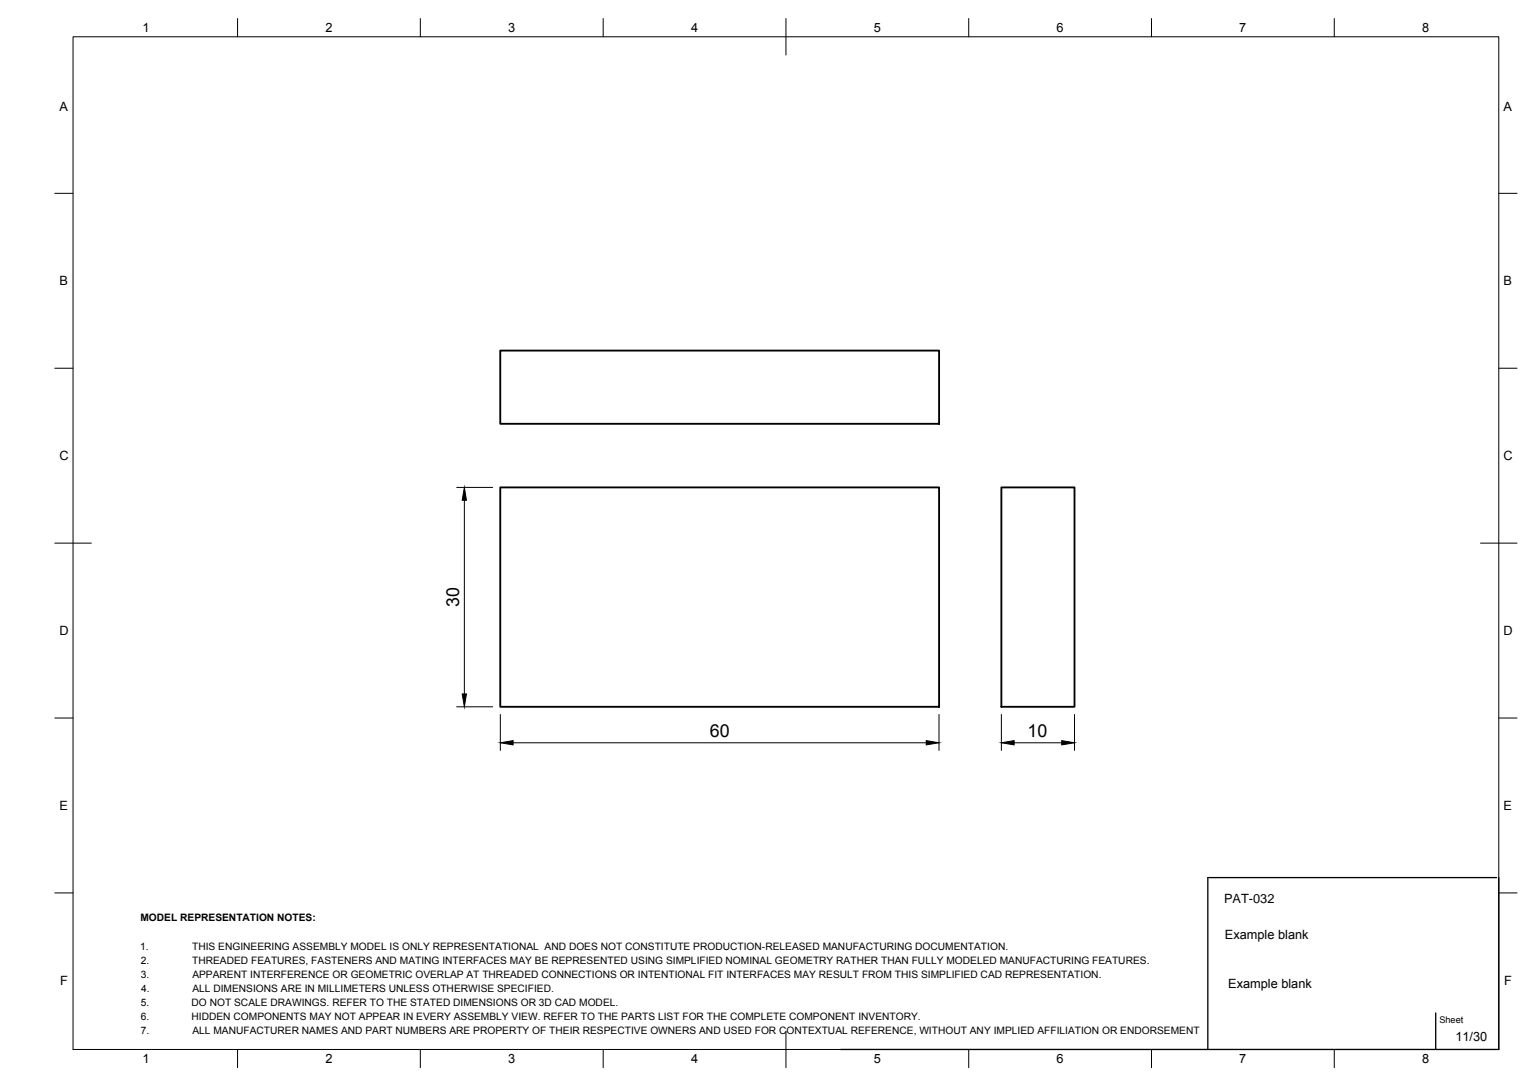
ISO-10303-21;
HEADER;
/* Generated by software containing ST-Developer
 * from STEP Tools, Inc. (www.steptools.com) 
 */

FILE_DESCRIPTION(
/* description */ ('Drill jig with bushing plate'),
/* implementation_level */ '2;1');

FILE_NAME(
/* name */ 'Example blank.step',
/* time_stamp */ '2026-10-27T10:51:08-07:00',
/* author */ (''),
/* organization */ (''),
/* preprocessor_version */ 'ST-DEVELOPER v20.2',
/* originating_system */ 'Autodesk Translation Framework v15.17.0.0',
/* authorisation */ '');

FILE_SCHEMA (('AUTOMOTIVE_DESIGN { 1 0 10303 214 3 1 1 }'));
ENDSEC;

DATA;
#10=MECHANICAL_DESIGN_GEOMETRIC_PRESENTATION_REPRESENTATION('',(#229),#6638);
#181=SHAPE_REPRESENTATION_RELATIONSHIP('SRR','None',#6745,#205);
#205=ADVANCED_BREP_SHAPE_REPRESENTATION('',(#253),#6618);
#229=STYLED_ITEM('',(#6929),#253);
#253=MANIFOLD_SOLID_BREP('Body1',#3596);
#399=PLANE('',#3997);
#400=PLANE('',#3998);
#401=PLANE('',#3999);
#402=PLANE('',#4000);
#403=PLANE('',#4001);
#404=PLANE('',#4002);
#556=FACE_OUTER_BOUND('',#811,.T.);
#557=FACE_OUTER_BOUND('',#812,.T.);
#558=FACE_OUTER_BOUND('',#813,.T.);
#559=FACE_OUTER_BOUND('',#814,.T.);
#560=FACE_OUTER_BOUND('',#815,.T.);
#561=FACE_OUTER_BOUND('',#816,.T.);
#811=EDGE_LOOP('',(#2665,#2666,#2667,#2668));
#812=EDGE_LOOP('',(#2669,#2670,#2671,#2672));
#813=EDGE_LOOP('',(#2673,#2674,#2675,#2676));
#814=EDGE_LOOP('',(#2677,#2678,#2679,#2680));
#815=EDGE_LOOP('',(#2681,#2682,#2683,#2684));
#816=EDGE_LOOP('',(#2685,#2686,#2687,#2688));
#1092=LINE('',#5743,#1353);
#1093=LINE('',#5745,#1354);
#1094=LINE('',#5747,#1355);
#1095=LINE('',#5748,#1356);
#1096=LINE('',#5751,#1357);
#1097=LINE('',#5753,#1358);
#1098=LINE('',#5754,#1359);
#1099=LINE('',#5757,#1360);
#1100=LINE('',#5759,#1361);
#1101=LINE('',#5760,#1362);
#1102=LINE('',#5762,#1363);
#1103=LINE('',#5763,#1364);
#1353=VECTOR('',#4625,1.);
#1354=VECTOR('',#4626,1.);
#1355=VECTOR('',#4627,1.);
#1356=VECTOR('',#4628,1.);
#1357=VECTOR('',#4631,1.);
#1358=VECTOR('',#4632,1.);
#1359=VECTOR('',#4633,1.);
#1360=VECTOR('',#4636,1.);
#1361=VECTOR('',#4637,1.);
#1362=VECTOR('',#4638,1.);
#1363=VECTOR('',#4641,1.);
#1364=VECTOR('',#4642,1.);
#1796=VERTEX_POINT('',#5741);
#1797=VERTEX_POINT('',#5742);
#1798=VERTEX_POINT('',#5744);
#1799=VERTEX_POINT('',#5746);
#1800=VERTEX_POINT('',#5750);
#1801=VERTEX_POINT('',#5752);
#1802=VERTEX_POINT('',#5756);
#1803=VERTEX_POINT('',#5758);
#2120=EDGE_CURVE('',#1796,#1797,#1092,.T.);
#2121=EDGE_CURVE('',#1797,#1798,#1093,.T.);
#2122=EDGE_CURVE('',#1799,#1798,#1094,.T.);
#2123=EDGE_CURVE('',#1796,#1799,#1095,.T.);
#2124=EDGE_CURVE('',#1800,#1796,#1096,.T.);
#2125=EDGE_CURVE('',#1801,#1799,#1097,.T.);
#2126=EDGE_CURVE('',#1800,#1801,#1098,.T.);
#2127=EDGE_CURVE('',#1802,#1800,#1099,.T.);
#2128=EDGE_CURVE('',#1803,#1801,#1100,.T.);
#2129=EDGE_CURVE('',#1802,#1803,#1101,.T.);
#2130=EDGE_CURVE('',#1797,#1802,#1102,.T.);
#2131=EDGE_CURVE('',#1798,#1803,#1103,.T.);
#2665=ORIENTED_EDGE('',*,*,#2120,.T.);
#2666=ORIENTED_EDGE('',*,*,#2121,.T.);
#2667=ORIENTED_EDGE('',*,*,#2122,.F.);
#2668=ORIENTED_EDGE('',*,*,#2123,.F.);
#2669=ORIENTED_EDGE('',*,*,#2124,.T.);
#2670=ORIENTED_EDGE('',*,*,#2123,.T.);
#2671=ORIENTED_EDGE('',*,*,#2125,.F.);
#2672=ORIENTED_EDGE('',*,*,#2126,.F.);
#2673=ORIENTED_EDGE('',*,*,#2127,.T.);
#2674=ORIENTED_EDGE('',*,*,#2126,.T.);
#2675=ORIENTED_EDGE('',*,*,#2128,.F.);
#2676=ORIENTED_EDGE('',*,*,#2129,.F.);
#2677=ORIENTED_EDGE('',*,*,#2130,.T.);
#2678=ORIENTED_EDGE('',*,*,#2129,.T.);
#2679=ORIENTED_EDGE('',*,*,#2131,.F.);
#2680=ORIENTED_EDGE('',*,*,#2121,.F.);
#2681=ORIENTED_EDGE('',*,*,#2131,.T.);
#2682=ORIENTED_EDGE('',*,*,#2128,.T.);
#2683=ORIENTED_EDGE('',*,*,#2125,.T.);
#2684=ORIENTED_EDGE('',*,*,#2122,.T.);
#2685=ORIENTED_EDGE('',*,*,#2130,.F.);
#2686=ORIENTED_EDGE('',*,*,#2120,.F.);
#2687=ORIENTED_EDGE('',*,*,#2124,.F.);
#2688=ORIENTED_EDGE('',*,*,#2127,.F.);
#3431=ADVANCED_FACE('',(#556),#399,.T.);
#3432=ADVANCED_FACE('',(#557),#400,.T.);
#3433=ADVANCED_FACE('',(#558),#401,.T.);
#3434=ADVANCED_FACE('',(#559),#402,.T.);
#3435=ADVANCED_FACE('',(#560),#403,.T.);
#3436=ADVANCED_FACE('',(#561),#404,.F.);
#3596=CLOSED_SHELL('',(#3431,#3432,#3433,#3434,#3435,#3436));
#3996=AXIS2_PLACEMENT_3D('',#5739,#4621,#4622);
#3997=AXIS2_PLACEMENT_3D('',#5740,#4623,#4624);
#3998=AXIS2_PLACEMENT_3D('',#5749,#4629,#4630);
#3999=AXIS2_PLACEMENT_3D('',#5755,#4634,#4635);
#4000=AXIS2_PLACEMENT_3D('',#5761,#4639,#4640);
#4001=AXIS2_PLACEMENT_3D('',#5764,#4643,#4644);
#4002=AXIS2_PLACEMENT_3D('',#5765,#4645,#4646);
#4621=DIRECTION('axis',(0.,0.,1.));
#4622=DIRECTION('refdir',(1.,0.,0.));
#4623=DIRECTION('center_axis',(0.,1.,0.));
#4624=DIRECTION('ref_axis',(-1.,0.,0.));
#4625=DIRECTION('',(-1.,0.,0.));
#4626=DIRECTION('',(0.,0.,1.));
#4627=DIRECTION('',(-1.,0.,0.));
#4628=DIRECTION('',(0.,0.,1.));
#4629=DIRECTION('center_axis',(1.,0.,0.));
#4630=DIRECTION('ref_axis',(0.,1.,0.));
#4631=DIRECTION('',(0.,1.,0.));
#4632=DIRECTION('',(0.,1.,0.));
#4633=DIRECTION('',(0.,0.,1.));
#4634=DIRECTION('center_axis',(0.,-1.,0.));
#4635=DIRECTION('ref_axis',(1.,0.,0.));
#4636=DIRECTION('',(1.,0.,0.));
#4637=DIRECTION('',(1.,0.,0.));
#4638=DIRECTION('',(0.,0.,1.));
#4639=DIRECTION('center_axis',(-1.,0.,0.));
#4640=DIRECTION('ref_axis',(0.,-1.,0.));
#4641=DIRECTION('',(0.,-1.,0.));
#4642=DIRECTION('',(0.,-1.,0.));
#4643=DIRECTION('center_axis',(0.,0.,1.));
#4644=DIRECTION('ref_axis',(1.,0.,0.));
#4645=DIRECTION('center_axis',(0.,0.,1.));
#4646=DIRECTION('ref_axis',(1.,0.,0.));
#5739=CARTESIAN_POINT('',(0.,0.,0.));
#5740=CARTESIAN_POINT('Origin',(3.,1.5,1.5));
#5741=CARTESIAN_POINT('',(3.,1.5,1.5));
#5742=CARTESIAN_POINT('',(-3.,1.5,1.5));
#5743=CARTESIAN_POINT('',(3.,1.5,1.5));
#5744=CARTESIAN_POINT('',(-3.,1.5,2.5));
#5745=CARTESIAN_POINT('',(-3.,1.5,1.5));
#5746=CARTESIAN_POINT('',(3.,1.5,2.5));
#5747=CARTESIAN_POINT('',(3.,1.5,2.5));
#5748=CARTESIAN_POINT('',(3.,1.5,1.5));
#5749=CARTESIAN_POINT('Origin',(3.,-1.5,1.5));
#5750=CARTESIAN_POINT('',(3.,-1.5,1.5));
#5751=CARTESIAN_POINT('',(3.,-1.5,1.5));
#5752=CARTESIAN_POINT('',(3.,-1.5,2.5));
#5753=CARTESIAN_POINT('',(3.,-1.5,2.5));
#5754=CARTESIAN_POINT('',(3.,-1.5,1.5));
#5755=CARTESIAN_POINT('Origin',(-3.,-1.5,1.5));
#5756=CARTESIAN_POINT('',(-3.,-1.5,1.5));
#5757=CARTESIAN_POINT('',(-3.,-1.5,1.5));
#5758=CARTESIAN_POINT('',(-3.,-1.5,2.5));
#5759=CARTESIAN_POINT('',(-3.,-1.5,2.5));
#5760=CARTESIAN_POINT('',(-3.,-1.5,1.5));
#5761=CARTESIAN_POINT('Origin',(-3.,1.5,1.5));
#5762=CARTESIAN_POINT('',(-3.,1.5,1.5));
#5763=CARTESIAN_POINT('',(-3.,1.5,2.5));
#5764=CARTESIAN_POINT('Origin',(0.,0.,2.5));
#5765=CARTESIAN_POINT('Origin',(0.,0.,1.5));
#6589=UNCERTAINTY_MEASURE_WITH_UNIT(LENGTH_MEASURE(0.001),#6639,
'DISTANCE_ACCURACY_VALUE',
'Maximum model space distance between geometric entities at asserted c
onnectivities');
#6609=UNCERTAINTY_MEASURE_WITH_UNIT(LENGTH_MEASURE(0.001),#6639,
'DISTANCE_ACCURACY_VALUE',
'Maximum model space distance between geometric entities at asserted c
onnectivities');
#6618=(
GEOMETRIC_REPRESENTATION_CONTEXT(3)
GLOBAL_UNCERTAINTY_ASSIGNED_CONTEXT((#6589))
GLOBAL_UNIT_ASSIGNED_CONTEXT((#6639,#6641,#6642))
REPRESENTATION_CONTEXT('','3D')
);
#6638=(
GEOMETRIC_REPRESENTATION_CONTEXT(3)
GLOBAL_UNCERTAINTY_ASSIGNED_CONTEXT((#6609))
GLOBAL_UNIT_ASSIGNED_CONTEXT((#6639,#6641,#6642))
REPRESENTATION_CONTEXT('','3D')
);
#6639=(
LENGTH_UNIT()
NAMED_UNIT(*)
SI_UNIT(.CENTI.,.METRE.)
);
#6641=(
NAMED_UNIT(*)
PLANE_ANGLE_UNIT()
SI_UNIT($,.RADIAN.)
);
#6642=(
NAMED_UNIT(*)
SI_UNIT($,.STERADIAN.)
SOLID_ANGLE_UNIT()
);
#6651=SHAPE_DEFINITION_REPRESENTATION(#6679,#6745);
#6679=PRODUCT_DEFINITION_SHAPE('',$,#6774);
#6745=SHAPE_REPRESENTATION('',(#3996),#6618);
#6765=PRODUCT_DEFINITION_CONTEXT('part definition',#6851,'design');
#6774=PRODUCT_DEFINITION('Example blank','Example blank',#6802,#6765);
#6802=PRODUCT_DEFINITION_FORMATION('',$,#6861);
#6851=APPLICATION_CONTEXT(
'Core Data for Automotive Mechanical Design Process');
#6852=PRODUCT_CONTEXT('part definition',#6851,'mechanical');
#6861=PRODUCT('Example blank','Example blank','Example blank',(#6852));
#6923=COLOUR_RGB('Light Blue',0.38,0.62,0.78);
#6924=FILL_AREA_STYLE_COLOUR('',#6923);
#6925=FILL_AREA_STYLE('',(#6924));
#6926=SURFACE_STYLE_FILL_AREA(#6925);
#6927=SURFACE_SIDE_STYLE('',(#6926));
#6928=SURFACE_STYLE_USAGE(.BOTH.,#6927);
#6929=PRESENTATION_STYLE_ASSIGNMENT((#6928));
ENDSEC;
END-ISO-10303-21;
